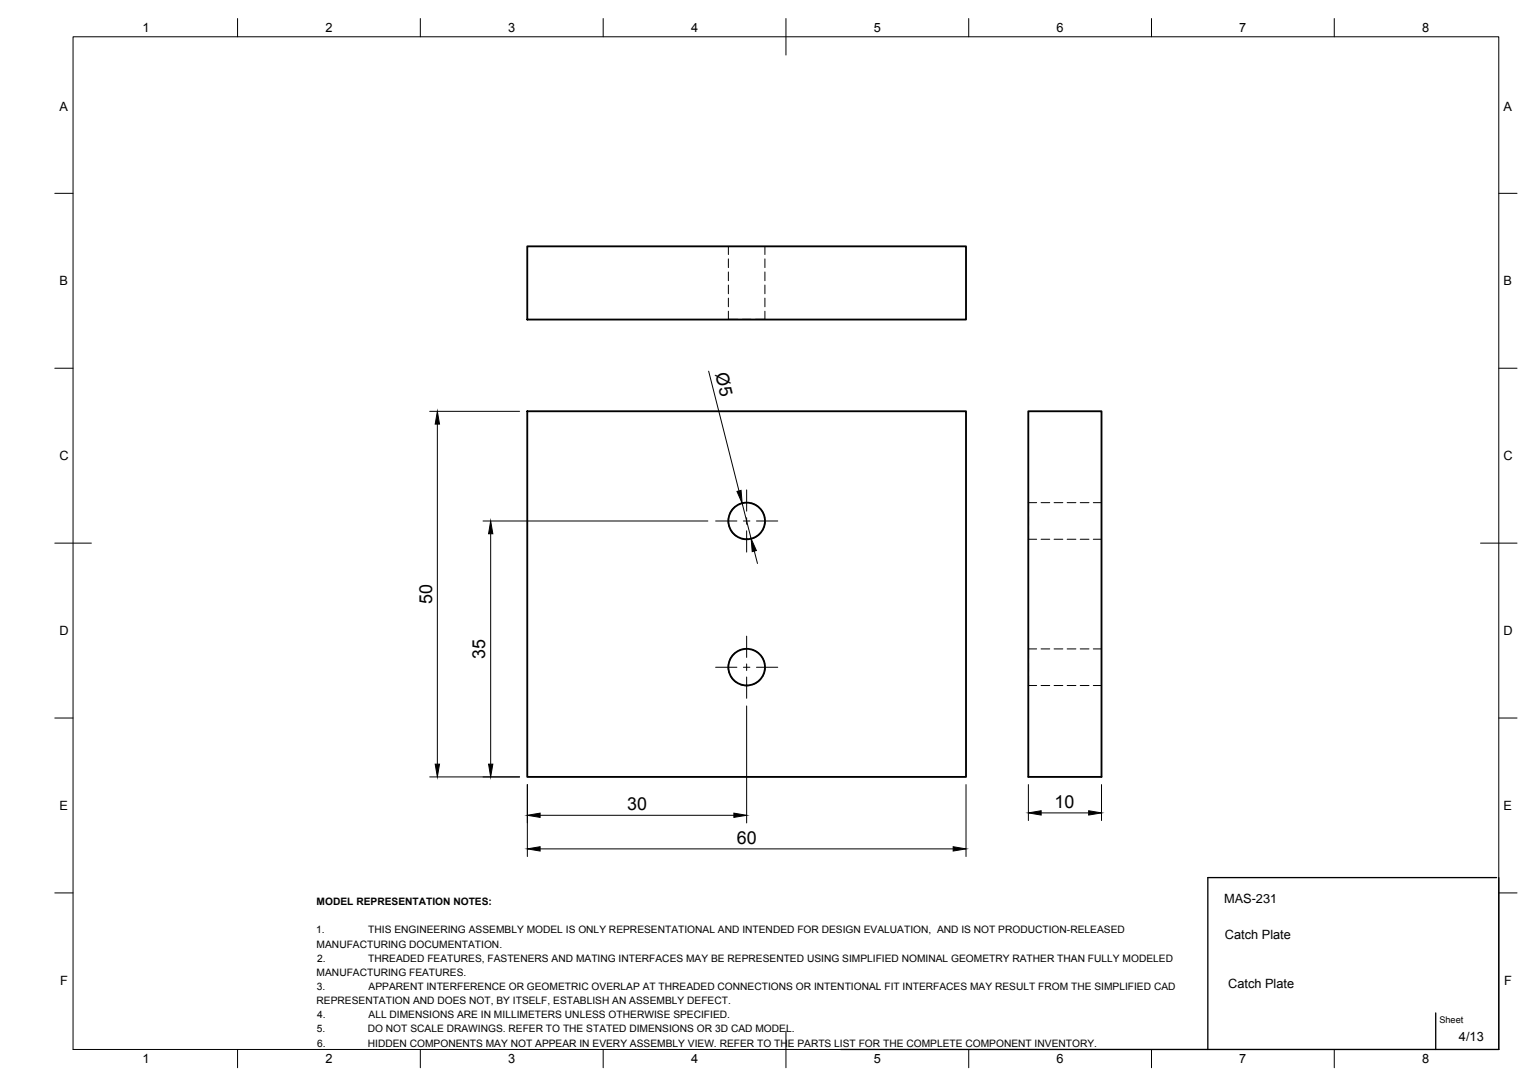
ISO-10303-21;
HEADER;
FILE_DESCRIPTION (('STEP AP214'),
    '1' );
FILE_NAME ( 'Catch Plate.step', '2026-10-04T02:08:54', ( '' ), ( '' ), 'STEP AP214', 'Unspecified', '' );
FILE_SCHEMA (( 'AUTOMOTIVE_DESIGN' ));
ENDSEC;
DATA;
#39=VERTEX_POINT ( 'NONE', #1053 ) ;
#195=CARTESIAN_POINT ( 'NONE',  ( -1.181102362204724310, 0.000000000000000000, 0.9842519685039370358 ) ) ;
#259=EDGE_CURVE ( 'NONE', #25443, #30394, #12521, .T. ) ;
#435=LINE ( 'NONE', #44275, #37021 ) ;
#465=DIRECTION ( 'NONE',  ( 0.000000000000000000, -1.000000000000000000, -0.000000000000000000 ) ) ;
#489=FACE_OUTER_BOUND ( 'NONE', #28194, .T. ) ;
#747=CARTESIAN_POINT ( 'NONE',  ( -1.181162989532618060E-16, -0.0009842519685041700977, -0.3937007874015748254 ) ) ;
#764=PLANE ( 'NONE',  #10375 ) ;
#918=CARTESIAN_POINT ( 'NONE',  ( 1.351300519334104211E-16, 0.000000000000000000, 0.2942913385826777528 ) ) ;
#939=CARTESIAN_POINT ( 'NONE',  ( 1.229559056033039366E-16, -0.3937007874015746034, 0.3937007874015748254 ) ) ;
#970=LINE ( 'NONE', #33143, #21182 ) ;
#1053=CARTESIAN_POINT ( 'NONE',  ( -1.181162989532618060E-16, 0.000000000000000000, -0.2942913385826778083 ) ) ;
#1089=AXIS2_PLACEMENT_3D ( 'NONE', #19982, #5124, #34384 ) ;
#1248=ORIENTED_EDGE ( 'NONE', *, *, #7894, .F. ) ;
#1492=LINE ( 'NONE', #22848, #24213 ) ;
#1504=APPLICATION_CONTEXT ( 'automotive_design' ) ;
#1636=DIRECTION ( 'NONE',  ( -0.000000000000000000, 1.000000000000000000, 0.000000000000000000 ) ) ;
#2032=ORIENTED_EDGE ( 'NONE', *, *, #20257, .F. ) ;
#2058=DIRECTION ( 'NONE',  ( 0.000000000000000000, 0.000000000000000000, 1.000000000000000000 ) ) ;
#2111=DIRECTION ( 'NONE',  ( 0.000000000000000000, -0.000000000000000000, 1.000000000000000000 ) ) ;
#2357=DIRECTION ( 'NONE',  ( -0.000000000000000000, 1.000000000000000000, -0.000000000000000000 ) ) ;
#2486=CONICAL_SURFACE ( 'NONE', #27822, 0.09842519685039320676, 0.7853981633972574317 ) ;
#2836=ORIENTED_EDGE ( 'NONE', *, *, #3131, .F. ) ;
#2971=LINE ( 'NONE', #28177, #16210 ) ;
#3019=VERTEX_POINT ( 'NONE', #18333 ) ;
#3116=CIRCLE ( 'NONE', #29957, 0.09842519685039317900 ) ;
#3131=EDGE_CURVE ( 'NONE', #40452, #34618, #3116, .T. ) ;
#3240=AXIS2_PLACEMENT_3D ( 'NONE', #24586, #9508, #14284 ) ;
#3282=DIRECTION ( 'NONE',  ( 0.000000000000000000, 1.000000000000000000, 0.000000000000000000 ) ) ;
#3475=DIRECTION ( 'NONE',  ( 0.000000000000000000, 0.000000000000000000, 1.000000000000000000 ) ) ;
#3902=CIRCLE ( 'NONE', #29213, 0.09842519685039317900 ) ;
#3961=ADVANCED_FACE ( 'NONE', ( #13385 ), #8628, .F. ) ;
#4097=DIRECTION ( 'NONE',  ( 0.000000000000000000, 0.000000000000000000, 1.000000000000000000 ) ) ;
#4138=FACE_BOUND ( 'NONE', #41382, .T. ) ;
#4204=PLANE ( 'NONE',  #12619 ) ;
#4433=CARTESIAN_POINT ( 'NONE',  ( 1.181102362204724310, 0.000000000000000000, -0.9842519685039370358 ) ) ;
#4439=DIRECTION ( 'NONE',  ( -0.000000000000000000, 1.000000000000000000, -0.000000000000000000 ) ) ;
#4522=DIRECTION ( 'NONE',  ( -0.000000000000000000, 1.000000000000000000, -0.000000000000000000 ) ) ;
#4677=SHAPE_REPRESENTATION ( 'Catch Plate', ( #20860 ), #39224 ) ;
#4714=AXIS2_PLACEMENT_3D ( 'NONE', #12097, #26721, #36779 ) ;
#5063=ORIENTED_EDGE ( 'NONE', *, *, #24553, .F. ) ;
#5124=DIRECTION ( 'NONE',  ( -0.000000000000000000, 1.000000000000000000, -0.000000000000000000 ) ) ;
#5226=VECTOR ( 'NONE', #25768, 39.37007874015748143 ) ;
#5569=DIRECTION ( 'NONE',  ( 0.000000000000000000, 0.000000000000000000, 1.000000000000000000 ) ) ;
#5636=ADVANCED_BREP_SHAPE_REPRESENTATION ( 'Catch Plate', ( #35488, #20860 ), #39224 ) ;
#5653=CARTESIAN_POINT ( 'NONE',  ( 1.229559056033039366E-16, 0.000000000000000000, 0.3937007874015748254 ) ) ;
#5807=ORIENTED_EDGE ( 'NONE', *, *, #22370, .F. ) ;
#6008=PRESENTATION_STYLE_ASSIGNMENT (( #9146 ) ) ;
#6027=DIRECTION ( 'NONE',  ( 0.000000000000000000, 1.000000000000000000, 0.000000000000000000 ) ) ;
#6152=PLANE ( 'NONE',  #43018 ) ;
#6237=( LENGTH_UNIT ( ) NAMED_UNIT ( * ) SI_UNIT ( $, .METRE. ) ) ;
#6272=DIMENSIONAL_EXPONENTS ( 1.000000000000000000, 0.000000000000000000, 0.000000000000000000, 0.000000000000000000, 0.000000000000000000, 0.000000000000000000, 0.000000000000000000 ) ;
#6313=STYLED_ITEM ( 'NONE', ( #6008 ), #35488 ) ;
#6328=AXIS2_PLACEMENT_3D ( 'NONE', #9787, #19060, #26758 ) ;
#6332=PRODUCT_DEFINITION ( 'UNKNOWN', '', #41536, #43673 ) ;
#6613=VERTEX_POINT ( 'NONE', #18873 ) ;
#6863=AXIS2_PLACEMENT_3D ( 'NONE', #39705, #10031, #36397 ) ;
#6997=CARTESIAN_POINT ( 'NONE',  ( 1.229559056033039366E-16, -0.0009842519685041700977, 0.4921259842519680183 ) ) ;
#7017=CIRCLE ( 'NONE', #10875, 0.09842519685039320676 ) ;
#7046=CARTESIAN_POINT ( 'NONE',  ( -1.181162989532618060E-16, 0.000000000000000000, -0.3937007874015748254 ) ) ;
#7141=UNCERTAINTY_MEASURE_WITH_UNIT (LENGTH_MEASURE( 1.000000000000000082E-05 ), #26155, 'distance_accuracy_value', 'NONE') ;
#7217=ORIENTED_EDGE ( 'NONE', *, *, #25255, .T. ) ;
#7258=CIRCLE ( 'NONE', #27942, 0.09940944881889700324 ) ;
#7304=LINE ( 'NONE', #21924, #46139 ) ;
#7465=CARTESIAN_POINT ( 'NONE',  ( -1.181162989532618060E-16, -0.0009842519685041700977, -0.3937007874015748254 ) ) ;
#7631=DIRECTION ( 'NONE',  ( 1.000000000000000000, 0.000000000000000000, 0.000000000000000000 ) ) ;
#7844=EDGE_CURVE ( 'NONE', #34120, #46098, #45511, .T. ) ;
#7855=CARTESIAN_POINT ( 'NONE',  ( -1.181162989532618060E-16, 0.000000000000000000, -0.3937007874015748254 ) ) ;
#7894=EDGE_CURVE ( 'NONE', #39, #44444, #7258, .T. ) ;
#8090=DIRECTION ( 'NONE',  ( -0.000000000000000000, 1.000000000000000000, -0.000000000000000000 ) ) ;
#8101=EDGE_CURVE ( 'NONE', #30394, #22319, #13184, .T. ) ;
#8152=ORIENTED_EDGE ( 'NONE', *, *, #18556, .F. ) ;
#8180=ORIENTED_EDGE ( 'NONE', *, *, #43386, .T. ) ;
#8546=CARTESIAN_POINT ( 'NONE',  ( 1.181102362204724310, -0.3937007874015748254, 0.9842519685039370358 ) ) ;
#8583=ORIENTED_EDGE ( 'NONE', *, *, #34147, .T. ) ;
#8628=CONICAL_SURFACE ( 'NONE', #6328, 0.09842519685039317900, 0.7853981633972921816 ) ;
#8637=DIRECTION ( 'NONE',  ( 0.000000000000000000, 0.000000000000000000, 1.000000000000000000 ) ) ;
#8713=LINE ( 'NONE', #31024, #47389 ) ;
#8717=CARTESIAN_POINT ( 'NONE',  ( 1.229559056033039366E-16, -0.0009842519685041700977, 0.3937007874015748254 ) ) ;
#8886=EDGE_CURVE ( 'NONE', #44444, #39, #34884, .T. ) ;
#8939=PRODUCT_CONTEXT ( 'NONE', #43789, 'mechanical' ) ;
#9029=EDGE_LOOP ( 'NONE', ( #32991, #10164, #38111, #16704 ) ) ;
#9146=SURFACE_STYLE_USAGE ( .BOTH. , #39067 ) ;
#9176=VECTOR ( 'NONE', #19339, 39.37007874015748143 ) ;
#9238=ADVANCED_FACE ( 'NONE', ( #18869 ), #29719, .F. ) ;
#9282=ADVANCED_FACE ( 'NONE', ( #40548, #4138, #18759 ), #764, .F. ) ;
#9508=DIRECTION ( 'NONE',  ( 0.000000000000000000, -1.000000000000000000, -0.000000000000000000 ) ) ;
#9655=VECTOR ( 'NONE', #24616, 39.37007874015748143 ) ;
#9761=ORIENTED_EDGE ( 'NONE', *, *, #34147, .F. ) ;
#9787=CARTESIAN_POINT ( 'NONE',  ( 1.229559056033039366E-16, -0.0009842519685041700977, 0.3937007874015748254 ) ) ;
#10012=LINE ( 'NONE', #14554, #44486 ) ;
#10031=DIRECTION ( 'NONE',  ( 0.000000000000000000, 1.000000000000000000, 0.000000000000000000 ) ) ;
#10164=ORIENTED_EDGE ( 'NONE', *, *, #8101, .T. ) ;
#10312=EDGE_LOOP ( 'NONE', ( #22832, #36137, #15653, #27504 ) ) ;
#10375=AXIS2_PLACEMENT_3D ( 'NONE', #11828, #26451, #37448 ) ;
#10570=AXIS2_PLACEMENT_3D ( 'NONE', #939, #4522, #33578 ) ;
#10660=CIRCLE ( 'NONE', #23649, 0.09842519685039317900 ) ;
#10761=CARTESIAN_POINT ( 'NONE',  ( -1.181102362204724310, 0.000000000000000000, -0.9842519685039370358 ) ) ;
#10835=DIRECTION ( 'NONE',  ( 1.000000000000000000, 0.000000000000000000, 0.000000000000000000 ) ) ;
#10875=AXIS2_PLACEMENT_3D ( 'NONE', #38399, #6027, #5569 ) ;
#10991=LINE ( 'NONE', #21760, #15302 ) ;
#11198=AXIS2_PLACEMENT_3D ( 'NONE', #43488, #21211, #28439 ) ;
#11292=ORIENTED_EDGE ( 'NONE', *, *, #7894, .T. ) ;
#11479=DIRECTION ( 'NONE',  ( 0.000000000000000000, 1.000000000000000000, 0.000000000000000000 ) ) ;
#11598=CARTESIAN_POINT ( 'NONE',  ( 1.229559056033039366E-16, 0.000000000000000000, 0.4931102362204718426 ) ) ;
#11620=CARTESIAN_POINT ( 'NONE',  ( -1.181162989532618060E-16, 0.000000000000000000, -0.2952755905511816326 ) ) ;
#11719=COLOUR_RGB ( '', 0.40784314, 0.44705882, 0.49803922) ;
#11828=CARTESIAN_POINT ( 'NONE',  ( 0.000000000000000000, -0.3937007874015748254, 0.000000000000000000 ) ) ;
#11952=PRODUCT_DEFINITION_SHAPE ( 'NONE', 'NONE',  #6332 ) ;
#11981=EDGE_CURVE ( 'NONE', #30394, #25443, #45738, .T. ) ;
#12097=CARTESIAN_POINT ( 'NONE',  ( 1.181102362204724310, -0.3937007874015748254, -0.9842519685039370358 ) ) ;
#12521=CIRCLE ( 'NONE', #1089, 0.09842519685039317900 ) ;
#12585=VERTEX_POINT ( 'NONE', #23013 ) ;
#12619=AXIS2_PLACEMENT_3D ( 'NONE', #19547, #37276, #26047 ) ;
#12653=ORIENTED_EDGE ( 'NONE', *, *, #35124, .F. ) ;
#12956=CARTESIAN_POINT ( 'NONE',  ( -1.181162989532618060E-16, 0.000000000000000000, -0.3937007874015748254 ) ) ;
#13022=SHAPE_DEFINITION_REPRESENTATION ( #11952, #4677 ) ;
#13149=CARTESIAN_POINT ( 'NONE',  ( 1.181102362204724310, -0.3937007874015748254, 0.9842519685039370358 ) ) ;
#13184=LINE ( 'NONE', #31633, #39386 ) ;
#13245=ORIENTED_EDGE ( 'NONE', *, *, #34990, .F. ) ;
#13385=FACE_OUTER_BOUND ( 'NONE', #29012, .T. ) ;
#13528=ORIENTED_EDGE ( 'NONE', *, *, #35124, .T. ) ;
#14038=FACE_OUTER_BOUND ( 'NONE', #17821, .T. ) ;
#14160=ORIENTED_EDGE ( 'NONE', *, *, #19162, .F. ) ;
#14284=DIRECTION ( 'NONE',  ( 0.000000000000000000, 0.000000000000000000, 1.000000000000000000 ) ) ;
#14554=CARTESIAN_POINT ( 'NONE',  ( 1.181102362204724310, -0.3937007874015748254, -0.9842519685039370358 ) ) ;
#14709=ORIENTED_EDGE ( 'NONE', *, *, #25221, .T. ) ;
#14956=EDGE_CURVE ( 'NONE', #12585, #22114, #28152, .T. ) ;
#14983=DIRECTION ( 'NONE',  ( -1.000000000000000000, 0.000000000000000000, 0.000000000000000000 ) ) ;
#15048=ORIENTED_EDGE ( 'NONE', *, *, #30836, .F. ) ;
#15302=VECTOR ( 'NONE', #21992, 39.37007874015748143 ) ;
#15367=EDGE_LOOP ( 'NONE', ( #39727, #43485 ) ) ;
#15578=CARTESIAN_POINT ( 'NONE',  ( -1.181102362204724310, -0.3937007874015748254, 0.9842519685039370358 ) ) ;
#15653=ORIENTED_EDGE ( 'NONE', *, *, #43594, .T. ) ;
#15790=CARTESIAN_POINT ( 'NONE',  ( 1.181102362204724310, 0.000000000000000000, 0.9842519685039370358 ) ) ;
#16096=CARTESIAN_POINT ( 'NONE',  ( 1.229559056033039366E-16, 0.000000000000000000, 0.3937007874015748254 ) ) ;
#16210=VECTOR ( 'NONE', #25280, 39.37007874015748143 ) ;
#16282=FACE_BOUND ( 'NONE', #24824, .T. ) ;
#16308=( GEOMETRIC_REPRESENTATION_CONTEXT ( 3 ) GLOBAL_UNCERTAINTY_ASSIGNED_CONTEXT ( ( #37360 ) ) GLOBAL_UNIT_ASSIGNED_CONTEXT ( ( #31442, #28313, #31914 ) ) REPRESENTATION_CONTEXT ( 'NONE', 'WORKASPACE' ) ) ;
#16403=DIRECTION ( 'NONE',  ( 0.000000000000000000, 1.000000000000000000, 0.000000000000000000 ) ) ;
#16419=ORIENTED_EDGE ( 'NONE', *, *, #259, .T. ) ;
#16519=ORIENTED_EDGE ( 'NONE', *, *, #43386, .F. ) ;
#16704=ORIENTED_EDGE ( 'NONE', *, *, #39706, .F. ) ;
#16724=DIRECTION ( 'NONE',  ( 1.000000000000000000, -0.000000000000000000, 0.000000000000000000 ) ) ;
#17270=ORIENTED_EDGE ( 'NONE', *, *, #8101, .F. ) ;
#17390=ORIENTED_EDGE ( 'NONE', *, *, #43700, .T. ) ;
#17453=ORIENTED_EDGE ( 'NONE', *, *, #14956, .T. ) ;
#17571=DIRECTION ( 'NONE',  ( -1.000000000000000000, 0.000000000000000000, 0.000000000000000000 ) ) ;
#17682=FACE_OUTER_BOUND ( 'NONE', #33318, .T. ) ;
#17821=EDGE_LOOP ( 'NONE', ( #46949, #41887, #36288, #17453 ) ) ;
#18333=CARTESIAN_POINT ( 'NONE',  ( 1.181102362204724310, -0.3937007874015748254, -0.9842519685039370358 ) ) ;
#18507=ORIENTED_EDGE ( 'NONE', *, *, #28425, .F. ) ;
#18556=EDGE_CURVE ( 'NONE', #3019, #25965, #10012, .T. ) ;
#18682=DIRECTION ( 'NONE',  ( 0.000000000000000000, 0.000000000000000000, 1.000000000000000000 ) ) ;
#18759=FACE_OUTER_BOUND ( 'NONE', #24238, .T. ) ;
#18790=PLANE ( 'NONE',  #4714 ) ;
#18869=FACE_OUTER_BOUND ( 'NONE', #40537, .T. ) ;
#18873=CARTESIAN_POINT ( 'NONE',  ( -1.181162989532618060E-16, -0.0009842519685041700977, -0.2952755905511816326 ) ) ;
#18945=DIRECTION ( 'NONE',  ( -0.000000000000000000, 1.000000000000000000, -0.000000000000000000 ) ) ;
#19060=DIRECTION ( 'NONE',  ( 0.000000000000000000, 1.000000000000000000, 0.000000000000000000 ) ) ;
#19162=EDGE_CURVE ( 'NONE', #21958, #44444, #2971, .T. ) ;
#19191=FACE_OUTER_BOUND ( 'NONE', #44539, .T. ) ;
#19339=DIRECTION ( 'NONE',  ( 0.000000000000000000, 1.000000000000000000, 0.000000000000000000 ) ) ;
#19369=ORIENTED_EDGE ( 'NONE', *, *, #39706, .T. ) ;
#19547=CARTESIAN_POINT ( 'NONE',  ( -1.181102362204724310, -0.3937007874015748254, 0.9842519685039370358 ) ) ;
#19610=LINE ( 'NONE', #41617, #33140 ) ;
#19982=CARTESIAN_POINT ( 'NONE',  ( 1.229559056033039366E-16, -0.3937007874015746034, 0.3937007874015748254 ) ) ;
#20113=VECTOR ( 'NONE', #45852, 39.37007874015748143 ) ;
#20257=EDGE_CURVE ( 'NONE', #31526, #22319, #3902, .T. ) ;
#20263=DIRECTION ( 'NONE',  ( -0.000000000000000000, 1.000000000000000000, -0.000000000000000000 ) ) ;
#20267=DIRECTION ( 'NONE',  ( 0.000000000000000000, 1.000000000000000000, 0.000000000000000000 ) ) ;
#20361=DIRECTION ( 'NONE',  ( 0.000000000000000000, -1.000000000000000000, -0.000000000000000000 ) ) ;
#20764=VECTOR ( 'NONE', #35646, 39.37007874015748143 ) ;
#20796=AXIS2_PLACEMENT_3D ( 'NONE', #7046, #33193, #46816 ) ;
#20860=AXIS2_PLACEMENT_3D ( 'NONE', #25692, #32652, #10835 ) ;
#21159=CARTESIAN_POINT ( 'NONE',  ( 1.181102362204724310, -0.3937007874015748254, -0.9842519685039370358 ) ) ;
#21182=VECTOR ( 'NONE', #30266, 39.37007874015748143 ) ;
#21211=DIRECTION ( 'NONE',  ( -1.000000000000000000, 0.000000000000000000, 0.000000000000000000 ) ) ;
#21482=LINE ( 'NONE', #28960, #9655 ) ;
#21705=DIRECTION ( 'NONE',  ( 0.000000000000000000, 1.000000000000000000, 0.000000000000000000 ) ) ;
#21760=CARTESIAN_POINT ( 'NONE',  ( 1.181102362204724310, 0.000000000000000000, 0.9842519685039370358 ) ) ;
#21924=CARTESIAN_POINT ( 'NONE',  ( 1.181102362204724310, 0.000000000000000000, -0.9842519685039370358 ) ) ;
#21958=VERTEX_POINT ( 'NONE', #25290 ) ;
#21992=DIRECTION ( 'NONE',  ( 0.000000000000000000, 0.000000000000000000, -1.000000000000000000 ) ) ;
#22114=VERTEX_POINT ( 'NONE', #30336 ) ;
#22134=ADVANCED_FACE ( 'NONE', ( #37240 ), #18790, .T. ) ;
#22278=DIRECTION ( 'NONE',  ( 0.000000000000000000, -1.000000000000000000, -0.000000000000000000 ) ) ;
#22319=VERTEX_POINT ( 'NONE', #34612 ) ;
#22370=EDGE_CURVE ( 'NONE', #22319, #31526, #35397, .T. ) ;
#22520=CARTESIAN_POINT ( 'NONE',  ( 1.229559056033039366E-16, 0.000000000000000000, 0.3937007874015748254 ) ) ;
#22538=LENGTH_MEASURE_WITH_UNIT ( LENGTH_MEASURE( 0.02539999999999999897 ), #36695 ) ;
#22812=DIRECTION ( 'NONE',  ( 0.000000000000000000, 0.000000000000000000, 1.000000000000000000 ) ) ;
#22832=ORIENTED_EDGE ( 'NONE', *, *, #30191, .F. ) ;
#22848=CARTESIAN_POINT ( 'NONE',  ( 1.181102362204724310, -0.3937007874015748254, 0.9842519685039370358 ) ) ;
#23013=CARTESIAN_POINT ( 'NONE',  ( -1.181102362204724310, -0.3937007874015748254, 0.9842519685039370358 ) ) ;
#23272=CYLINDRICAL_SURFACE ( 'NONE', #46359, 0.09842519685039317900 ) ;
#23372=ORIENTED_EDGE ( 'NONE', *, *, #7844, .F. ) ;
#23649=AXIS2_PLACEMENT_3D ( 'NONE', #26181, #32441, #36492 ) ;
#23835=ORIENTED_EDGE ( 'NONE', *, *, #259, .F. ) ;
#23871=FACE_OUTER_BOUND ( 'NONE', #9029, .T. ) ;
#23919=CIRCLE ( 'NONE', #3240, 0.09940944881889707263 ) ;
#23927=DIRECTION ( 'NONE',  ( 0.000000000000000000, 0.000000000000000000, 1.000000000000000000 ) ) ;
#24213=VECTOR ( 'NONE', #34357, 39.37007874015748143 ) ;
#24238=EDGE_LOOP ( 'NONE', ( #9761, #36887, #12653, #40782 ) ) ;
#24356=DIMENSIONAL_EXPONENTS ( 1.000000000000000000, 0.000000000000000000, 0.000000000000000000, 0.000000000000000000, 0.000000000000000000, 0.000000000000000000, 0.000000000000000000 ) ;
#24472=FILL_AREA_STYLE ('',( #28087 ) ) ;
#24553=EDGE_CURVE ( 'NONE', #25965, #30060, #7304, .T. ) ;
#24583=ORIENTED_EDGE ( 'NONE', *, *, #35619, .T. ) ;
#24586=CARTESIAN_POINT ( 'NONE',  ( 1.229559056033039366E-16, 0.000000000000000000, 0.3937007874015748254 ) ) ;
#24616=DIRECTION ( 'NONE',  ( -0.000000000000000000, 1.000000000000000000, -0.000000000000000000 ) ) ;
#24694=VECTOR ( 'NONE', #17571, 39.37007874015748143 ) ;
#24824=EDGE_LOOP ( 'NONE', ( #11292, #37537 ) ) ;
#25221=EDGE_CURVE ( 'NONE', #22114, #44500, #33070, .T. ) ;
#25255=EDGE_CURVE ( 'NONE', #30476, #44500, #435, .T. ) ;
#25280=DIRECTION ( 'NONE',  ( 8.659560562353279948E-17, 0.7071067811866824648, -0.7071067811864125696 ) ) ;
#25290=CARTESIAN_POINT ( 'NONE',  ( -1.060626887254335780E-16, -0.0009842519685041700977, -0.4921259842519680738 ) ) ;
#25439=VECTOR ( 'NONE', #36892, 39.37007874015748143 ) ;
#25443=VERTEX_POINT ( 'NONE', #34468 ) ;
#25692=CARTESIAN_POINT ( 'NONE',  ( 0.000000000000000000, 0.000000000000000000, 0.000000000000000000 ) ) ;
#25768=DIRECTION ( 'NONE',  ( -0.000000000000000000, 1.000000000000000000, -0.000000000000000000 ) ) ;
#25965=VERTEX_POINT ( 'NONE', #4433 ) ;
#26047=DIRECTION ( 'NONE',  ( 1.000000000000000000, 0.000000000000000000, -0.000000000000000000 ) ) ;
#26155=( CONVERSION_BASED_UNIT ( 'INCH', #22538 ) LENGTH_UNIT ( ) NAMED_UNIT ( #24356 ) ) ;
#26181=CARTESIAN_POINT ( 'NONE',  ( -1.181162989532618060E-16, -0.3937007874015746034, -0.3937007874015748254 ) ) ;
#26451=DIRECTION ( 'NONE',  ( -0.000000000000000000, 1.000000000000000000, 0.000000000000000000 ) ) ;
#26553=CARTESIAN_POINT ( 'NONE',  ( 1.350095158311321523E-16, -0.3937007874015746034, 0.2952755905511816326 ) ) ;
#26617=CARTESIAN_POINT ( 'NONE',  ( -1.181162989532618060E-16, 0.000000000000000000, -0.3937007874015748254 ) ) ;
#26721=DIRECTION ( 'NONE',  ( 0.000000000000000000, 0.000000000000000000, -1.000000000000000000 ) ) ;
#26758=DIRECTION ( 'NONE',  ( 0.000000000000000000, 0.000000000000000000, 1.000000000000000000 ) ) ;
#26847=CIRCLE ( 'NONE', #42088, 0.09842519685039320676 ) ;
#26850=EDGE_LOOP ( 'NONE', ( #32517, #41774, #8583, #7217 ) ) ;
#27504=ORIENTED_EDGE ( 'NONE', *, *, #18556, .T. ) ;
#27736=LINE ( 'NONE', #42302, #34523 ) ;
#27822=AXIS2_PLACEMENT_3D ( 'NONE', #747, #44597, #22812 ) ;
#27837=ORIENTED_EDGE ( 'NONE', *, *, #28166, .T. ) ;
#27942=AXIS2_PLACEMENT_3D ( 'NONE', #26617, #465, #41172 ) ;
#28087=FILL_AREA_STYLE_COLOUR ( '', #11719 ) ;
#28152=LINE ( 'NONE', #39138, #9176 ) ;
#28166=EDGE_CURVE ( 'NONE', #40452, #6613, #44405, .T. ) ;
#28177=CARTESIAN_POINT ( 'NONE',  ( -1.060626887254335780E-16, -0.0009842519685041700977, -0.4921259842519680183 ) ) ;
#28194=EDGE_LOOP ( 'NONE', ( #17270, #23835, #19369, #37306 ) ) ;
#28313=( NAMED_UNIT ( * ) PLANE_ANGLE_UNIT ( ) SI_UNIT ( $, .RADIAN. ) ) ;
#28425=EDGE_CURVE ( 'NONE', #22319, #34120, #8713, .T. ) ;
#28439=DIRECTION ( 'NONE',  ( 0.000000000000000000, 0.000000000000000000, 1.000000000000000000 ) ) ;
#28472=FACE_OUTER_BOUND ( 'NONE', #10312, .T. ) ;
#28519=DIRECTION ( 'NONE',  ( 0.000000000000000000, 0.000000000000000000, 1.000000000000000000 ) ) ;
#28825=ORIENTED_EDGE ( 'NONE', *, *, #34990, .T. ) ;
#28826=EDGE_CURVE ( 'NONE', #34618, #40452, #10660, .T. ) ;
#28924=PLANE ( 'NONE',  #11198 ) ;
#28960=CARTESIAN_POINT ( 'NONE',  ( -1.060626887254335780E-16, 0.000000000000000000, -0.4921259842519680183 ) ) ;
#29012=EDGE_LOOP ( 'NONE', ( #5807, #32201, #39992, #13245 ) ) ;
#29025=ORIENTED_EDGE ( 'NONE', *, *, #11981, .T. ) ;
#29213=AXIS2_PLACEMENT_3D ( 'NONE', #38947, #20267, #2058 ) ;
#29263=CARTESIAN_POINT ( 'NONE',  ( -1.059421526231553215E-16, 0.000000000000000000, -0.4931102362204718426 ) ) ;
#29285=LINE ( 'NONE', #15578, #25439 ) ;
#29557=SHAPE_REPRESENTATION_RELATIONSHIP ( 'NONE' , 'NONE' ,  #4677, #5636 ) ;
#29719=CYLINDRICAL_SURFACE ( 'NONE', #33352, 0.09842519685039320676 ) ;
#29920=DIRECTION ( 'NONE',  ( 0.000000000000000000, 0.000000000000000000, 1.000000000000000000 ) ) ;
#29957=AXIS2_PLACEMENT_3D ( 'NONE', #37285, #4439, #29920 ) ;
#30024=ADVANCED_FACE ( 'NONE', ( #17682 ), #39757, .F. ) ;
#30060=VERTEX_POINT ( 'NONE', #10761 ) ;
#30191=EDGE_CURVE ( 'NONE', #44500, #25965, #10991, .T. ) ;
#30228=ORIENTED_EDGE ( 'NONE', *, *, #45276, .T. ) ;
#30266=DIRECTION ( 'NONE',  ( -0.000000000000000000, 1.000000000000000000, -0.000000000000000000 ) ) ;
#30318=CARTESIAN_POINT ( 'NONE',  ( -1.181102362204724310, -0.3937007874015748254, -0.9842519685039370358 ) ) ;
#30336=CARTESIAN_POINT ( 'NONE',  ( -1.181102362204724310, 0.000000000000000000, 0.9842519685039370358 ) ) ;
#30394=VERTEX_POINT ( 'NONE', #26553 ) ;
#30476=VERTEX_POINT ( 'NONE', #8546 ) ;
#30813=LINE ( 'NONE', #38444, #20113 ) ;
#30817=EDGE_LOOP ( 'NONE', ( #14709, #38447, #46269, #24583 ) ) ;
#30836=EDGE_CURVE ( 'NONE', #6613, #21958, #26847, .T. ) ;
#30917=ORIENTED_EDGE ( 'NONE', *, *, #30836, .T. ) ;
#31024=CARTESIAN_POINT ( 'NONE',  ( 1.350095158311321523E-16, -0.0009842519685041700977, 0.2952755905511816326 ) ) ;
#31029=DIRECTION ( 'NONE',  ( 0.000000000000000000, 0.000000000000000000, 1.000000000000000000 ) ) ;
#31092=VECTOR ( 'NONE', #37704, 39.37007874015748143 ) ;
#31358=DIRECTION ( 'NONE',  ( 0.000000000000000000, 0.000000000000000000, -1.000000000000000000 ) ) ;
#31442=( CONVERSION_BASED_UNIT ( 'INCH', #35505 ) LENGTH_UNIT ( ) NAMED_UNIT ( #6272 ) ) ;
#31526=VERTEX_POINT ( 'NONE', #6997 ) ;
#31633=CARTESIAN_POINT ( 'NONE',  ( 1.350095158311321523E-16, 0.000000000000000000, 0.2952755905511816326 ) ) ;
#31914=( NAMED_UNIT ( * ) SI_UNIT ( $, .STERADIAN. ) SOLID_ANGLE_UNIT ( ) ) ;
#32201=ORIENTED_EDGE ( 'NONE', *, *, #28425, .T. ) ;
#32226=ADVANCED_FACE ( 'NONE', ( #23871 ), #35140, .F. ) ;
#32273=EDGE_CURVE ( 'NONE', #44530, #12585, #27736, .T. ) ;
#32302=LINE ( 'NONE', #34942, #20764 ) ;
#32441=DIRECTION ( 'NONE',  ( -0.000000000000000000, 1.000000000000000000, -0.000000000000000000 ) ) ;
#32517=ORIENTED_EDGE ( 'NONE', *, *, #25221, .F. ) ;
#32652=DIRECTION ( 'NONE',  ( 0.000000000000000000, 0.000000000000000000, 1.000000000000000000 ) ) ;
#32714=FACE_OUTER_BOUND ( 'NONE', #35242, .T. ) ;
#32991=ORIENTED_EDGE ( 'NONE', *, *, #11981, .F. ) ;
#33070=LINE ( 'NONE', #195, #46173 ) ;
#33140=VECTOR ( 'NONE', #23927, 39.37007874015748143 ) ;
#33143=CARTESIAN_POINT ( 'NONE',  ( 1.229559056033039366E-16, 0.000000000000000000, 0.4921259842519680183 ) ) ;
#33193=DIRECTION ( 'NONE',  ( -0.000000000000000000, 1.000000000000000000, -0.000000000000000000 ) ) ;
#33318=EDGE_LOOP ( 'NONE', ( #18507, #2032, #28825, #23372 ) ) ;
#33352=AXIS2_PLACEMENT_3D ( 'NONE', #7855, #8090, #33774 ) ;
#33578=DIRECTION ( 'NONE',  ( 0.000000000000000000, 0.000000000000000000, 1.000000000000000000 ) ) ;
#33633=FACE_OUTER_BOUND ( 'NONE', #43436, .T. ) ;
#33774=DIRECTION ( 'NONE',  ( 0.000000000000000000, 0.000000000000000000, 1.000000000000000000 ) ) ;
#34120=VERTEX_POINT ( 'NONE', #918 ) ;
#34147=EDGE_CURVE ( 'NONE', #12585, #30476, #29285, .T. ) ;
#34285=ADVANCED_FACE ( 'NONE', ( #16282, #45711, #37841 ), #45954, .T. ) ;
#34357=DIRECTION ( 'NONE',  ( 0.000000000000000000, 0.000000000000000000, -1.000000000000000000 ) ) ;
#34384=DIRECTION ( 'NONE',  ( 0.000000000000000000, 0.000000000000000000, 1.000000000000000000 ) ) ;
#34468=CARTESIAN_POINT ( 'NONE',  ( 1.229559056033039366E-16, -0.3937007874015746034, 0.4921259842519680183 ) ) ;
#34523=VECTOR ( 'NONE', #3475, 39.37007874015748143 ) ;
#34580=EDGE_CURVE ( 'NONE', #46098, #34120, #23919, .T. ) ;
#34607=DIRECTION ( 'NONE',  ( 8.659560562353580701E-17, 0.7071067811866579289, -0.7071067811864371055 ) ) ;
#34612=CARTESIAN_POINT ( 'NONE',  ( 1.350095158311321523E-16, -0.0009842519685041700977, 0.2952755905511816326 ) ) ;
#34618=VERTEX_POINT ( 'NONE', #35616 ) ;
#34807=SURFACE_STYLE_FILL_AREA ( #24472 ) ;
#34884=CIRCLE ( 'NONE', #40172, 0.09940944881889700324 ) ;
#34910=DIRECTION ( 'NONE',  ( 0.000000000000000000, 0.000000000000000000, 1.000000000000000000 ) ) ;
#34942=CARTESIAN_POINT ( 'NONE',  ( -1.181162989532618060E-16, -0.0009842519685041700977, -0.2952755905511816326 ) ) ;
#34967=CARTESIAN_POINT ( 'NONE',  ( 0.000000000000000000, 0.000000000000000000, 0.000000000000000000 ) ) ;
#34971=AXIS2_PLACEMENT_3D ( 'NONE', #7465, #40278, #4097 ) ;
#34990=EDGE_CURVE ( 'NONE', #31526, #46098, #30813, .T. ) ;
#35124=EDGE_CURVE ( 'NONE', #3019, #44530, #39366, .T. ) ;
#35140=CYLINDRICAL_SURFACE ( 'NONE', #46746, 0.09842519685039317900 ) ;
#35242=EDGE_LOOP ( 'NONE', ( #16519, #2836, #27837, #30917 ) ) ;
#35397=CIRCLE ( 'NONE', #36179, 0.09842519685039317900 ) ;
#35468=ADVANCED_FACE ( 'NONE', ( #33633 ), #2486, .F. ) ;
#35469=CLOSED_SHELL ( 'NONE', ( #3961, #39636, #32226, #9238, #41092, #38899, #22134, #46934, #9282, #34285, #45974, #39375, #35468, #30024 ) ) ;
#35470=ORIENTED_EDGE ( 'NONE', *, *, #46352, .F. ) ;
#35488=MANIFOLD_SOLID_BREP ( 'Catch Plate', #35469 ) ;
#35505=LENGTH_MEASURE_WITH_UNIT ( LENGTH_MEASURE( 0.02539999999999999897 ), #6237 ) ;
#35616=CARTESIAN_POINT ( 'NONE',  ( -1.060626887254335780E-16, -0.3937007874015746034, -0.4921259842519680183 ) ) ;
#35619=EDGE_CURVE ( 'NONE', #30060, #22114, #19610, .T. ) ;
#35646=DIRECTION ( 'NONE',  ( 0.000000000000000000, 0.7071067811866824648, 0.7071067811864125696 ) ) ;
#36048=CYLINDRICAL_SURFACE ( 'NONE', #20796, 0.09842519685039320676 ) ;
#36137=ORIENTED_EDGE ( 'NONE', *, *, #25255, .F. ) ;
#36152=ORIENTED_EDGE ( 'NONE', *, *, #19162, .T. ) ;
#36179=AXIS2_PLACEMENT_3D ( 'NONE', #8717, #16403, #31029 ) ;
#36288=ORIENTED_EDGE ( 'NONE', *, *, #32273, .T. ) ;
#36339=CARTESIAN_POINT ( 'NONE',  ( -1.181162989532618060E-16, -0.0009842519685041700977, -0.3937007874015748254 ) ) ;
#36354=AXIS2_PLACEMENT_3D ( 'NONE', #22520, #22278, #18682 ) ;
#36397=DIRECTION ( 'NONE',  ( 0.000000000000000000, 0.000000000000000000, 1.000000000000000000 ) ) ;
#36468=( NAMED_UNIT ( * ) PLANE_ANGLE_UNIT ( ) SI_UNIT ( $, .RADIAN. ) ) ;
#36492=DIRECTION ( 'NONE',  ( 0.000000000000000000, 0.000000000000000000, 1.000000000000000000 ) ) ;
#36695=( LENGTH_UNIT ( ) NAMED_UNIT ( * ) SI_UNIT ( $, .METRE. ) ) ;
#36771=CARTESIAN_POINT ( 'NONE',  ( -1.181162989532618060E-16, -0.3937007874015746034, -0.2952755905511816326 ) ) ;
#36779=DIRECTION ( 'NONE',  ( -1.000000000000000000, 0.000000000000000000, -0.000000000000000000 ) ) ;
#36887=ORIENTED_EDGE ( 'NONE', *, *, #32273, .F. ) ;
#36892=DIRECTION ( 'NONE',  ( 1.000000000000000000, 0.000000000000000000, 0.000000000000000000 ) ) ;
#36942=MECHANICAL_DESIGN_GEOMETRIC_PRESENTATION_REPRESENTATION('',(#6313),#16308);
#37021=VECTOR ( 'NONE', #11479, 39.37007874015748143 ) ;
#37157=ORIENTED_EDGE ( 'NONE', *, *, #46352, .T. ) ;
#37240=FACE_OUTER_BOUND ( 'NONE', #46939, .T. ) ;
#37276=DIRECTION ( 'NONE',  ( 0.000000000000000000, 0.000000000000000000, 1.000000000000000000 ) ) ;
#37285=CARTESIAN_POINT ( 'NONE',  ( -1.181162989532618060E-16, -0.3937007874015746034, -0.3937007874015748254 ) ) ;
#37306=ORIENTED_EDGE ( 'NONE', *, *, #20257, .T. ) ;
#37360=UNCERTAINTY_MEASURE_WITH_UNIT (LENGTH_MEASURE( 1.000000000000000082E-05 ), #31442, 'distance_accuracy_value', 'NONE') ;
#37448=DIRECTION ( 'NONE',  ( 0.000000000000000000, -0.000000000000000000, 1.000000000000000000 ) ) ;
#37523=FACE_OUTER_BOUND ( 'NONE', #26850, .T. ) ;
#37537=ORIENTED_EDGE ( 'NONE', *, *, #8886, .T. ) ;
#37565=CARTESIAN_POINT ( 'NONE',  ( -1.181102362204724310, -0.3937007874015748254, -0.9842519685039370358 ) ) ;
#37704=DIRECTION ( 'NONE',  ( 0.000000000000000000, 1.000000000000000000, 0.000000000000000000 ) ) ;
#37841=FACE_OUTER_BOUND ( 'NONE', #30817, .T. ) ;
#38111=ORIENTED_EDGE ( 'NONE', *, *, #22370, .T. ) ;
#38399=CARTESIAN_POINT ( 'NONE',  ( -1.181162989532618060E-16, -0.0009842519685041700977, -0.3937007874015748254 ) ) ;
#38444=CARTESIAN_POINT ( 'NONE',  ( 1.229559056033039366E-16, -0.0009842519685041700977, 0.4921259842519680183 ) ) ;
#38447=ORIENTED_EDGE ( 'NONE', *, *, #30191, .T. ) ;
#38899=ADVANCED_FACE ( 'NONE', ( #14038 ), #28924, .T. ) ;
#38947=CARTESIAN_POINT ( 'NONE',  ( 1.229559056033039366E-16, -0.0009842519685041700977, 0.3937007874015748254 ) ) ;
#39067=SURFACE_SIDE_STYLE ('',( #34807 ) ) ;
#39138=CARTESIAN_POINT ( 'NONE',  ( -1.181102362204724310, -0.3937007874015748254, 0.9842519685039370358 ) ) ;
#39224=( GEOMETRIC_REPRESENTATION_CONTEXT ( 3 ) GLOBAL_UNCERTAINTY_ASSIGNED_CONTEXT ( ( #7141 ) ) GLOBAL_UNIT_ASSIGNED_CONTEXT ( ( #26155, #36468, #40727 ) ) REPRESENTATION_CONTEXT ( 'NONE', 'WORKASPACE' ) ) ;
#39366=LINE ( 'NONE', #21159, #24694 ) ;
#39375=ADVANCED_FACE ( 'NONE', ( #489 ), #23272, .F. ) ;
#39386=VECTOR ( 'NONE', #2357, 39.37007874015748143 ) ;
#39636=ADVANCED_FACE ( 'NONE', ( #19191 ), #44875, .F. ) ;
#39705=CARTESIAN_POINT ( 'NONE',  ( 1.229559056033039366E-16, -0.0009842519685041700977, 0.3937007874015748254 ) ) ;
#39706=EDGE_CURVE ( 'NONE', #25443, #31526, #970, .T. ) ;
#39727=ORIENTED_EDGE ( 'NONE', *, *, #34580, .T. ) ;
#39757=CONICAL_SURFACE ( 'NONE', #6863, 0.09842519685039317900, 0.7853981633972921816 ) ;
#39992=ORIENTED_EDGE ( 'NONE', *, *, #34580, .F. ) ;
#40172=AXIS2_PLACEMENT_3D ( 'NONE', #12956, #20361, #28519 ) ;
#40278=DIRECTION ( 'NONE',  ( 0.000000000000000000, 1.000000000000000000, 0.000000000000000000 ) ) ;
#40452=VERTEX_POINT ( 'NONE', #36771 ) ;
#40537=EDGE_LOOP ( 'NONE', ( #42494, #8180, #37157, #41671 ) ) ;
#40548=FACE_BOUND ( 'NONE', #46373, .T. ) ;
#40727=( NAMED_UNIT ( * ) SI_UNIT ( $, .STERADIAN. ) SOLID_ANGLE_UNIT ( ) ) ;
#40782=ORIENTED_EDGE ( 'NONE', *, *, #43594, .F. ) ;
#41092=ADVANCED_FACE ( 'NONE', ( #37523 ), #4204, .T. ) ;
#41172=DIRECTION ( 'NONE',  ( 0.000000000000000000, 0.000000000000000000, 1.000000000000000000 ) ) ;
#41185=ORIENTED_EDGE ( 'NONE', *, *, #45276, .F. ) ;
#41382=EDGE_LOOP ( 'NONE', ( #45305, #45922 ) ) ;
#41536=PRODUCT_DEFINITION_FORMATION_WITH_SPECIFIED_SOURCE ( 'ANY', '', #44040, .NOT_KNOWN. ) ;
#41617=CARTESIAN_POINT ( 'NONE',  ( -1.181102362204724310, 0.000000000000000000, -0.9842519685039370358 ) ) ;
#41671=ORIENTED_EDGE ( 'NONE', *, *, #28166, .F. ) ;
#41774=ORIENTED_EDGE ( 'NONE', *, *, #14956, .F. ) ;
#41887=ORIENTED_EDGE ( 'NONE', *, *, #43700, .F. ) ;
#42088=AXIS2_PLACEMENT_3D ( 'NONE', #36339, #21705, #46852 ) ;
#42205=ORIENTED_EDGE ( 'NONE', *, *, #8886, .F. ) ;
#42302=CARTESIAN_POINT ( 'NONE',  ( -1.181102362204724310, -0.3937007874015748254, -0.9842519685039370358 ) ) ;
#42494=ORIENTED_EDGE ( 'NONE', *, *, #28826, .F. ) ;
#43018=AXIS2_PLACEMENT_3D ( 'NONE', #13149, #16724, #31358 ) ;
#43386=EDGE_CURVE ( 'NONE', #34618, #21958, #21482, .T. ) ;
#43436=EDGE_LOOP ( 'NONE', ( #14160, #15048, #30228, #42205 ) ) ;
#43485=ORIENTED_EDGE ( 'NONE', *, *, #7844, .T. ) ;
#43488=CARTESIAN_POINT ( 'NONE',  ( -1.181102362204724310, -0.3937007874015748254, -0.9842519685039370358 ) ) ;
#43594=EDGE_CURVE ( 'NONE', #30476, #3019, #1492, .T. ) ;
#43673=PRODUCT_DEFINITION_CONTEXT ( 'detailed design', #1504, 'design' ) ;
#43700=EDGE_CURVE ( 'NONE', #44530, #30060, #44625, .T. ) ;
#43789=APPLICATION_CONTEXT ( 'automotive_design' ) ;
#44040=PRODUCT ( 'Catch Plate', 'Catch Plate', '', ( #8939 ) ) ;
#44275=CARTESIAN_POINT ( 'NONE',  ( 1.181102362204724310, -0.3937007874015748254, 0.9842519685039370358 ) ) ;
#44405=LINE ( 'NONE', #11620, #5226 ) ;
#44444=VERTEX_POINT ( 'NONE', #29263 ) ;
#44486=VECTOR ( 'NONE', #3282, 39.37007874015748143 ) ;
#44500=VERTEX_POINT ( 'NONE', #15790 ) ;
#44530=VERTEX_POINT ( 'NONE', #37565 ) ;
#44539=EDGE_LOOP ( 'NONE', ( #35470, #36152, #1248, #41185 ) ) ;
#44597=DIRECTION ( 'NONE',  ( 0.000000000000000000, 1.000000000000000000, 0.000000000000000000 ) ) ;
#44625=LINE ( 'NONE', #30318, #31092 ) ;
#44875=CONICAL_SURFACE ( 'NONE', #34971, 0.09842519685039320676, 0.7853981633972574317 ) ;
#45276=EDGE_CURVE ( 'NONE', #6613, #39, #32302, .T. ) ;
#45303=AXIS2_PLACEMENT_3D ( 'NONE', #34967, #1636, #2111 ) ;
#45305=ORIENTED_EDGE ( 'NONE', *, *, #3131, .T. ) ;
#45511=CIRCLE ( 'NONE', #36354, 0.09940944881889707263 ) ;
#45711=FACE_BOUND ( 'NONE', #15367, .T. ) ;
#45738=CIRCLE ( 'NONE', #10570, 0.09842519685039317900 ) ;
#45852=DIRECTION ( 'NONE',  ( 0.000000000000000000, 0.7071067811866579289, 0.7071067811864371055 ) ) ;
#45922=ORIENTED_EDGE ( 'NONE', *, *, #28826, .T. ) ;
#45954=PLANE ( 'NONE',  #45303 ) ;
#45974=ADVANCED_FACE ( 'NONE', ( #32714 ), #36048, .F. ) ;
#46098=VERTEX_POINT ( 'NONE', #11598 ) ;
#46139=VECTOR ( 'NONE', #14983, 39.37007874015748143 ) ;
#46173=VECTOR ( 'NONE', #7631, 39.37007874015748143 ) ;
#46269=ORIENTED_EDGE ( 'NONE', *, *, #24553, .T. ) ;
#46352=EDGE_CURVE ( 'NONE', #21958, #6613, #7017, .T. ) ;
#46359=AXIS2_PLACEMENT_3D ( 'NONE', #16096, #18945, #8637 ) ;
#46373=EDGE_LOOP ( 'NONE', ( #16419, #29025 ) ) ;
#46746=AXIS2_PLACEMENT_3D ( 'NONE', #5653, #20263, #34910 ) ;
#46816=DIRECTION ( 'NONE',  ( 0.000000000000000000, 0.000000000000000000, 1.000000000000000000 ) ) ;
#46852=DIRECTION ( 'NONE',  ( 0.000000000000000000, 0.000000000000000000, 1.000000000000000000 ) ) ;
#46934=ADVANCED_FACE ( 'NONE', ( #28472 ), #6152, .T. ) ;
#46939=EDGE_LOOP ( 'NONE', ( #5063, #8152, #13528, #17390 ) ) ;
#46949=ORIENTED_EDGE ( 'NONE', *, *, #35619, .F. ) ;
#47389=VECTOR ( 'NONE', #34607, 39.37007874015748143 ) ;
ENDSEC;
END-ISO-10303-21;
